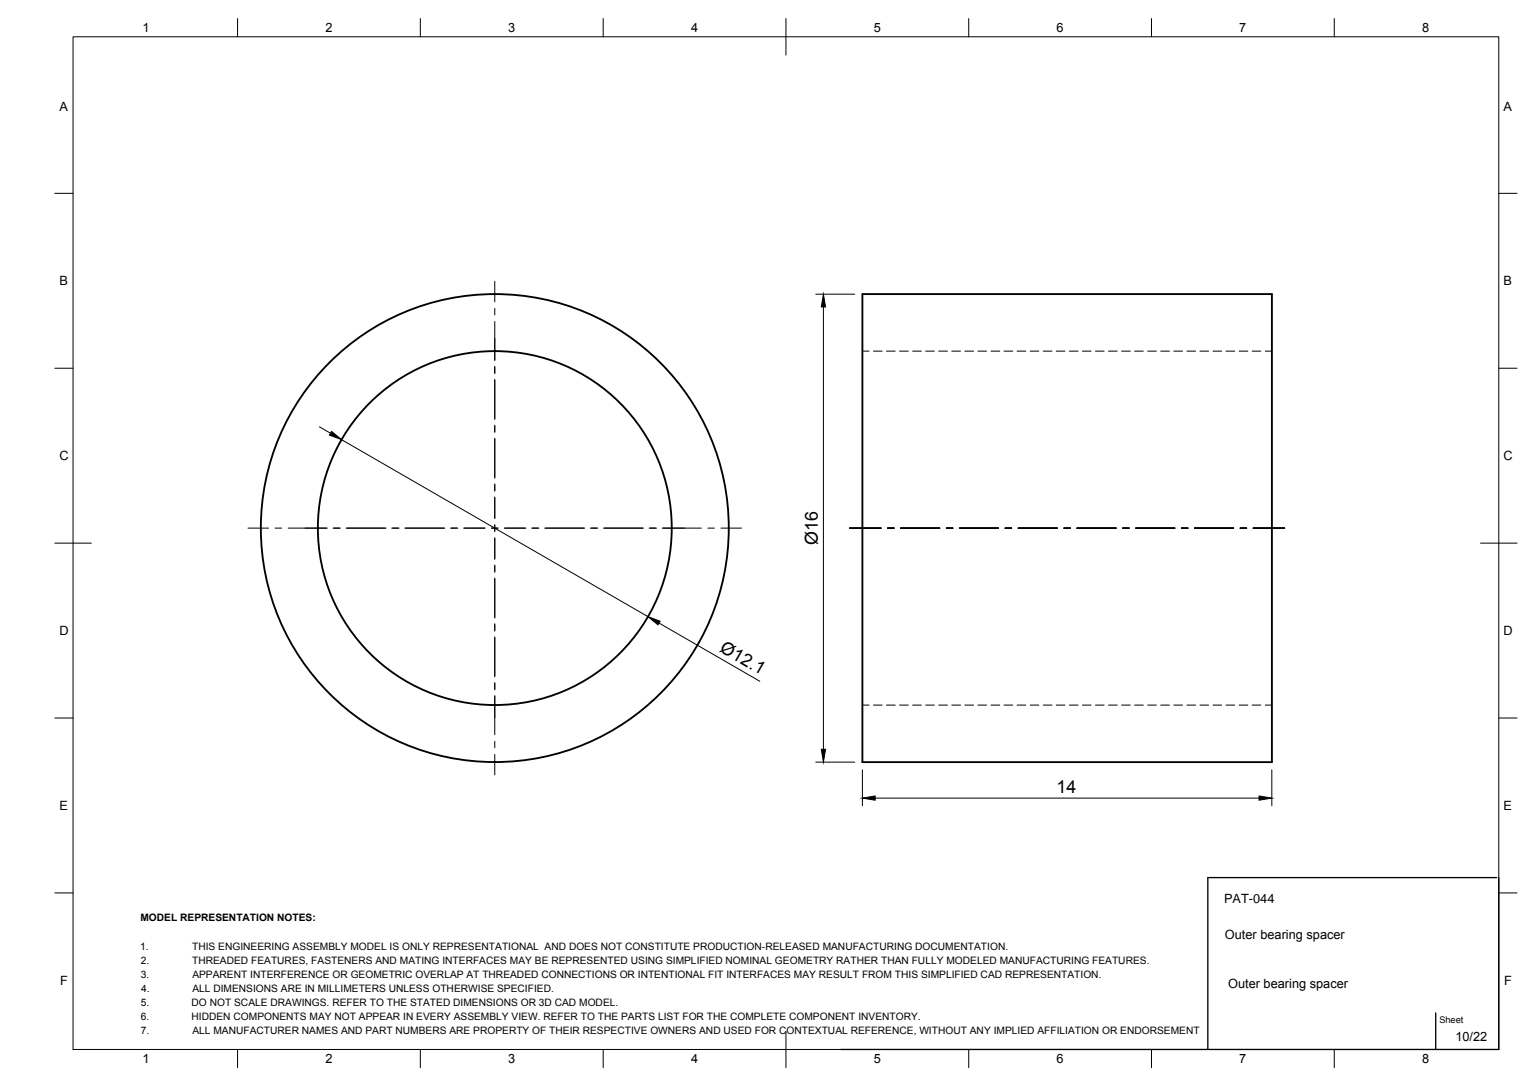
ISO-10303-21;
HEADER;
/* Generated by software containing ST-Developer
 * from STEP Tools, Inc. (www.steptools.com) 
 */

FILE_DESCRIPTION(
/* description */ ('Four-wheel beam trolley'),
/* implementation_level */ '2;1');

FILE_NAME(
/* name */ 'Outer bearing spacer.step',
/* time_stamp */ '2026-10-29T16:22:06-07:00',
/* author */ (''),
/* organization */ (''),
/* preprocessor_version */ 'ST-DEVELOPER v20.2',
/* originating_system */ 'Autodesk Translation Framework v15.17.0.0',
/* authorisation */ '');

FILE_SCHEMA (('AUTOMOTIVE_DESIGN { 1 0 10303 214 3 1 1 }'));
ENDSEC;

DATA;
#10=MECHANICAL_DESIGN_GEOMETRIC_PRESENTATION_REPRESENTATION('',(#285),#4777);
#251=SHAPE_REPRESENTATION_RELATIONSHIP('SRR','None',#4880,#268);
#268=ADVANCED_BREP_SHAPE_REPRESENTATION('',(#308),#4765);
#285=STYLED_ITEM('',(#5056),#308);
#308=MANIFOLD_SOLID_BREP('Body1',#2373);
#345=FACE_BOUND('',#676,.T.);
#346=FACE_BOUND('',#678,.T.);
#405=PLANE('',#2700);
#406=PLANE('',#2701);
#505=FACE_OUTER_BOUND('',#673,.T.);
#506=FACE_OUTER_BOUND('',#674,.T.);
#507=FACE_OUTER_BOUND('',#675,.T.);
#508=FACE_OUTER_BOUND('',#677,.T.);
#673=EDGE_LOOP('',(#1857,#1858,#1859,#1860));
#674=EDGE_LOOP('',(#1861,#1862,#1863,#1864));
#675=EDGE_LOOP('',(#1865));
#676=EDGE_LOOP('',(#1866));
#677=EDGE_LOOP('',(#1867));
#678=EDGE_LOOP('',(#1868));
#851=LINE('',#4030,#974);
#852=LINE('',#4036,#975);
#974=VECTOR('',#3240,0.605);
#975=VECTOR('',#3247,0.8);
#1065=CIRCLE('',#2695,0.605);
#1066=CIRCLE('',#2696,0.605);
#1067=CIRCLE('',#2698,0.8);
#1068=CIRCLE('',#2699,0.8);
#1237=VERTEX_POINT('',#4027);
#1238=VERTEX_POINT('',#4029);
#1239=VERTEX_POINT('',#4033);
#1240=VERTEX_POINT('',#4035);
#1466=EDGE_CURVE('',#1237,#1237,#1065,.T.);
#1467=EDGE_CURVE('',#1237,#1238,#851,.T.);
#1468=EDGE_CURVE('',#1238,#1238,#1066,.T.);
#1469=EDGE_CURVE('',#1239,#1239,#1067,.T.);
#1470=EDGE_CURVE('',#1239,#1240,#852,.T.);
#1471=EDGE_CURVE('',#1240,#1240,#1068,.T.);
#1857=ORIENTED_EDGE('',*,*,#1466,.F.);
#1858=ORIENTED_EDGE('',*,*,#1467,.T.);
#1859=ORIENTED_EDGE('',*,*,#1468,.T.);
#1860=ORIENTED_EDGE('',*,*,#1467,.F.);
#1861=ORIENTED_EDGE('',*,*,#1469,.F.);
#1862=ORIENTED_EDGE('',*,*,#1470,.T.);
#1863=ORIENTED_EDGE('',*,*,#1471,.T.);
#1864=ORIENTED_EDGE('',*,*,#1470,.F.);
#1865=ORIENTED_EDGE('',*,*,#1469,.T.);
#1866=ORIENTED_EDGE('',*,*,#1466,.T.);
#1867=ORIENTED_EDGE('',*,*,#1471,.F.);
#1868=ORIENTED_EDGE('',*,*,#1468,.F.);
#2194=CYLINDRICAL_SURFACE('',#2694,0.605);
#2195=CYLINDRICAL_SURFACE('',#2697,0.8);
#2281=ADVANCED_FACE('',(#505),#2194,.F.);
#2282=ADVANCED_FACE('',(#506),#2195,.T.);
#2283=ADVANCED_FACE('',(#507,#345),#405,.T.);
#2284=ADVANCED_FACE('',(#508,#346),#406,.F.);
#2373=CLOSED_SHELL('',(#2281,#2282,#2283,#2284));
#2693=AXIS2_PLACEMENT_3D('',#4025,#3234,#3235);
#2694=AXIS2_PLACEMENT_3D('',#4026,#3236,#3237);
#2695=AXIS2_PLACEMENT_3D('',#4028,#3238,#3239);
#2696=AXIS2_PLACEMENT_3D('',#4031,#3241,#3242);
#2697=AXIS2_PLACEMENT_3D('',#4032,#3243,#3244);
#2698=AXIS2_PLACEMENT_3D('',#4034,#3245,#3246);
#2699=AXIS2_PLACEMENT_3D('',#4037,#3248,#3249);
#2700=AXIS2_PLACEMENT_3D('',#4038,#3250,#3251);
#2701=AXIS2_PLACEMENT_3D('',#4039,#3252,#3253);
#3234=DIRECTION('axis',(0.,0.,1.));
#3235=DIRECTION('refdir',(1.,0.,0.));
#3236=DIRECTION('center_axis',(0.,1.,0.));
#3237=DIRECTION('ref_axis',(1.,0.,0.));
#3238=DIRECTION('center_axis',(0.,-1.,0.));
#3239=DIRECTION('ref_axis',(1.,0.,0.));
#3240=DIRECTION('',(0.,-1.,0.));
#3241=DIRECTION('center_axis',(0.,-1.,0.));
#3242=DIRECTION('ref_axis',(1.,0.,0.));
#3243=DIRECTION('center_axis',(0.,1.,0.));
#3244=DIRECTION('ref_axis',(1.,0.,0.));
#3245=DIRECTION('center_axis',(0.,1.,0.));
#3246=DIRECTION('ref_axis',(1.,0.,0.));
#3247=DIRECTION('',(0.,-1.,0.));
#3248=DIRECTION('center_axis',(0.,1.,0.));
#3249=DIRECTION('ref_axis',(1.,0.,0.));
#3250=DIRECTION('center_axis',(0.,1.,0.));
#3251=DIRECTION('ref_axis',(1.,0.,0.));
#3252=DIRECTION('center_axis',(0.,1.,0.));
#3253=DIRECTION('ref_axis',(1.,0.,0.));
#4025=CARTESIAN_POINT('',(0.,0.,0.));
#4026=CARTESIAN_POINT('Origin',(0.,4.1,13.75));
#4027=CARTESIAN_POINT('',(-0.605,5.5,13.75));
#4028=CARTESIAN_POINT('Origin',(0.,5.5,13.75));
#4029=CARTESIAN_POINT('',(-0.605,4.1,13.75));
#4030=CARTESIAN_POINT('',(-0.605,4.1,13.75));
#4031=CARTESIAN_POINT('Origin',(0.,4.1,13.75));
#4032=CARTESIAN_POINT('Origin',(0.,4.1,13.75));
#4033=CARTESIAN_POINT('',(-0.8,5.5,13.75));
#4034=CARTESIAN_POINT('Origin',(0.,5.5,13.75));
#4035=CARTESIAN_POINT('',(-0.8,4.1,13.75));
#4036=CARTESIAN_POINT('',(-0.8,4.1,13.75));
#4037=CARTESIAN_POINT('Origin',(0.,4.1,13.75));
#4038=CARTESIAN_POINT('Origin',(0.,5.5,13.75));
#4039=CARTESIAN_POINT('Origin',(0.,4.1,13.75));
#4743=UNCERTAINTY_MEASURE_WITH_UNIT(LENGTH_MEASURE(0.001),#4778,
'DISTANCE_ACCURACY_VALUE',
'Maximum model space distance between geometric entities at asserted c
onnectivities');
#4755=UNCERTAINTY_MEASURE_WITH_UNIT(LENGTH_MEASURE(0.001),#4778,
'DISTANCE_ACCURACY_VALUE',
'Maximum model space distance between geometric entities at asserted c
onnectivities');
#4765=(
GEOMETRIC_REPRESENTATION_CONTEXT(3)
GLOBAL_UNCERTAINTY_ASSIGNED_CONTEXT((#4743))
GLOBAL_UNIT_ASSIGNED_CONTEXT((#4778,#4780,#4781))
REPRESENTATION_CONTEXT('','3D')
);
#4777=(
GEOMETRIC_REPRESENTATION_CONTEXT(3)
GLOBAL_UNCERTAINTY_ASSIGNED_CONTEXT((#4755))
GLOBAL_UNIT_ASSIGNED_CONTEXT((#4778,#4780,#4781))
REPRESENTATION_CONTEXT('','3D')
);
#4778=(
LENGTH_UNIT()
NAMED_UNIT(*)
SI_UNIT(.CENTI.,.METRE.)
);
#4780=(
NAMED_UNIT(*)
PLANE_ANGLE_UNIT()
SI_UNIT($,.RADIAN.)
);
#4781=(
NAMED_UNIT(*)
SI_UNIT($,.STERADIAN.)
SOLID_ANGLE_UNIT()
);
#4791=SHAPE_DEFINITION_REPRESENTATION(#4812,#4880);
#4812=PRODUCT_DEFINITION_SHAPE('',$,#4902);
#4880=SHAPE_REPRESENTATION('',(#2693),#4765);
#4892=PRODUCT_DEFINITION_CONTEXT('part definition',#4957,'design');
#4902=PRODUCT_DEFINITION('Outer bearing spacer','Outer bearing spacer',
#4923,#4892);
#4923=PRODUCT_DEFINITION_FORMATION('',$,#4968);
#4957=APPLICATION_CONTEXT(
'Core Data for Automotive Mechanical Design Process');
#4958=PRODUCT_CONTEXT('part definition',#4957,'mechanical');
#4968=PRODUCT('Outer bearing spacer','Outer bearing spacer',
'Outer bearing spacer',(#4958));
#5050=COLOUR_RGB('Grey',0.48,0.52,0.57);
#5051=FILL_AREA_STYLE_COLOUR('',#5050);
#5052=FILL_AREA_STYLE('',(#5051));
#5053=SURFACE_STYLE_FILL_AREA(#5052);
#5054=SURFACE_SIDE_STYLE('',(#5053));
#5055=SURFACE_STYLE_USAGE(.BOTH.,#5054);
#5056=PRESENTATION_STYLE_ASSIGNMENT((#5055));
ENDSEC;
END-ISO-10303-21;
